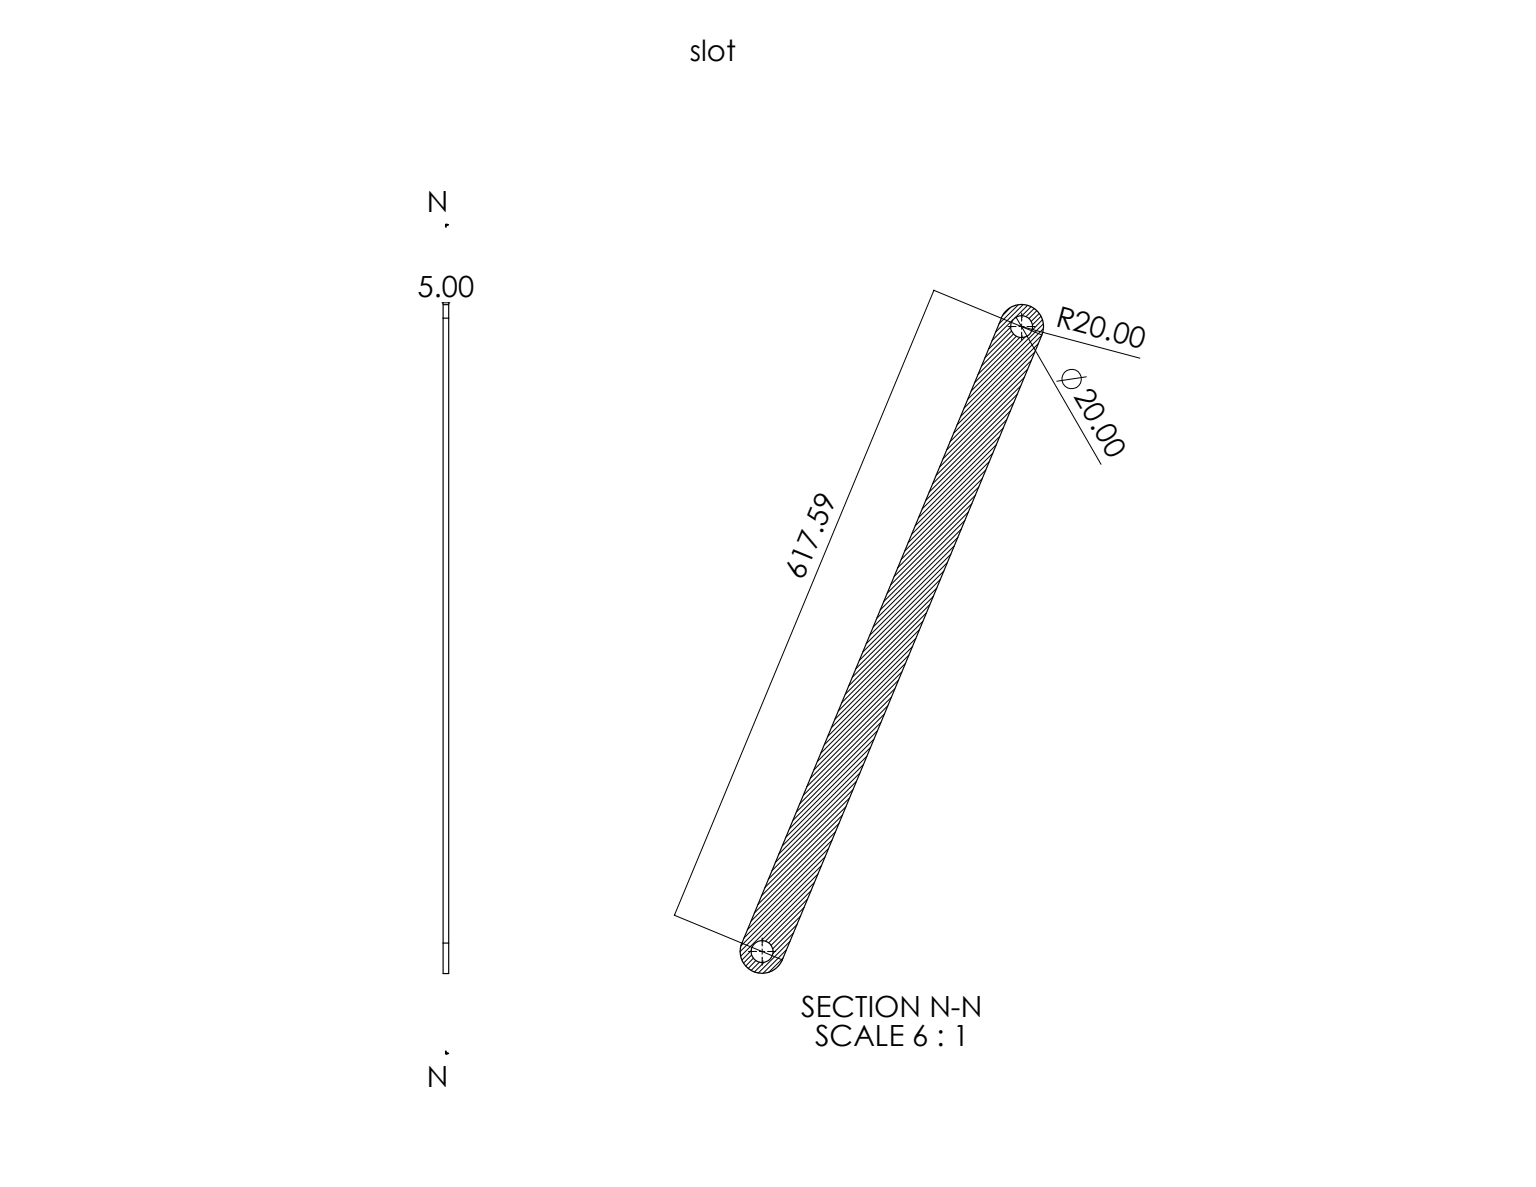
ISO-10303-21;
HEADER;
FILE_DESCRIPTION (('STEP AP214'),
    '1' );
FILE_NAME ('Slot.step',
    '2026-10-21T17:07:05',
    ( '' ),
    ( '' ),
    'SwSTEP 2.0',
    'SolidWorks 2025',
    '' );
FILE_SCHEMA (( 'AUTOMOTIVE_DESIGN' ));
ENDSEC;

DATA;
#41=DIRECTION ( 'NONE',  ( 1.000000000000000000, 0.000000000000000000, 0.000000000000000000 ) ) ;
#52=CYLINDRICAL_SURFACE ( 'NONE', #32876, 9.999999999999980460 ) ;
#346=VERTEX_POINT ( 'NONE', #30093 ) ;
#367=EDGE_LOOP ( 'NONE', ( #42116, #38302, #12349, #11045 ) ) ;
#472=ORIENTED_EDGE ( 'NONE', *, *, #31485, .F. ) ;
#592=ORIENTED_EDGE ( 'NONE', *, *, #31485, .T. ) ;
#799=EDGE_LOOP ( 'NONE', ( #25522, #592, #42461, #2264, #39166 ) ) ;
#822=CARTESIAN_POINT ( 'NONE',  ( 799.9999999999993179, 205.0000000000000568, -255.0000000000000000 ) ) ;
#930=CIRCLE ( 'NONE', #36312, 10.00000000000000888 ) ;
#1035=CIRCLE ( 'NONE', #26827, 20.00000000000004619 ) ;
#1068=VECTOR ( 'NONE', #44629, 1000.000000000000000 ) ;
#1080=EDGE_LOOP ( 'NONE', ( #33357, #6990 ) ) ;
#1302=DIRECTION ( 'NONE',  ( 1.000000000000000000, 0.000000000000000000, 0.000000000000000000 ) ) ;
#1372=DIRECTION ( 'NONE',  ( 0.000000000000000000, 0.000000000000000000, -1.000000000000000000 ) ) ;
#1425=ORIENTED_EDGE ( 'NONE', *, *, #20505, .T. ) ;
#1710=CYLINDRICAL_SURFACE ( 'NONE', #21162, 9.999999999999982236 ) ;
#1788=EDGE_CURVE ( 'NONE', #28471, #16704, #1035, .T. ) ;
#1790=VECTOR ( 'NONE', #5422, 1000.000000000000000 ) ;
#1945=DIRECTION ( 'NONE',  ( -1.000000000000000000, -0.000000000000000000, -0.000000000000000000 ) ) ;
#1955=EDGE_CURVE ( 'NONE', #29157, #346, #26860, .T. ) ;
#2029=ORIENTED_EDGE ( 'NONE', *, *, #37278, .F. ) ;
#2061=EDGE_CURVE ( 'NONE', #2904, #27191, #30531, .T. ) ;
#2125=CIRCLE ( 'NONE', #8059, 20.00000000000004619 ) ;
#2238=ORIENTED_EDGE ( 'NONE', *, *, #32386, .T. ) ;
#2241=DIRECTION ( 'NONE',  ( -1.000000000000000000, -0.000000000000000000, -0.000000000000000000 ) ) ;
#2264=ORIENTED_EDGE ( 'NONE', *, *, #37278, .T. ) ;
#2415=EDGE_CURVE ( 'NONE', #35075, #33515, #40175, .T. ) ;
#2494=LINE ( 'NONE', #37839, #35001 ) ;
#2512=CARTESIAN_POINT ( 'NONE',  ( 799.9999999999993179, 205.0000000000000568, -255.0000000000000000 ) ) ;
#2552=ORIENTED_EDGE ( 'NONE', *, *, #44509, .T. ) ;
#2733=DIRECTION ( 'NONE',  ( -1.000000000000000000, -0.000000000000000000, -0.000000000000000000 ) ) ;
#2774=DIRECTION ( 'NONE',  ( -1.000000000000000000, -0.000000000000000000, -0.000000000000000000 ) ) ;
#2904=VERTEX_POINT ( 'NONE', #22866 ) ;
#2983=FACE_OUTER_BOUND ( 'NONE', #799, .T. ) ;
#3048=CARTESIAN_POINT ( 'NONE',  ( 799.9999999999993179, -365.3551492539851893, -18.13243251470705886 ) ) ;
#3132=ORIENTED_EDGE ( 'NONE', *, *, #28735, .F. ) ;
#3295=CIRCLE ( 'NONE', #4026, 9.999999999999980460 ) ;
#3590=DIRECTION ( 'NONE',  ( -1.000000000000000000, -0.000000000000000000, -0.000000000000000000 ) ) ;
#4011=DIRECTION ( 'NONE',  ( 0.000000000000000000, 0.000000000000000000, 1.000000000000000000 ) ) ;
#4026=AXIS2_PLACEMENT_3D ( 'NONE', #19087, #1302, #25779 ) ;
#4037=VERTEX_POINT ( 'NONE', #18447 ) ;
#4474=CYLINDRICAL_SURFACE ( 'NONE', #18007, 9.999999999999980460 ) ;
#4695=DIRECTION ( 'NONE',  ( 1.000000000000000000, 0.000000000000000000, 0.000000000000000000 ) ) ;
#4728=AXIS2_PLACEMENT_3D ( 'NONE', #30831, #20871, #44925 ) ;
#4975=LINE ( 'NONE', #37049, #24120 ) ;
#5041=CARTESIAN_POINT ( 'NONE',  ( 799.9999999999993179, -365.3551492539851893, -18.13243251470705886 ) ) ;
#5166=UNCERTAINTY_MEASURE_WITH_UNIT (LENGTH_MEASURE( 1.000000000000000082E-05 ), #31589, 'distance_accuracy_value', 'NONE');
#5422=DIRECTION ( 'NONE',  ( -1.000000000000000000, -0.000000000000000000, -0.000000000000000000 ) ) ;
#5439=ORIENTED_EDGE ( 'NONE', *, *, #32681, .F. ) ;
#5952=LINE ( 'NONE', #12438, #14488 ) ;
#5959=CARTESIAN_POINT ( 'NONE',  ( 799.9999999999993179, -365.3551492539851893, -18.13243251470705886 ) ) ;
#5960=ORIENTED_EDGE ( 'NONE', *, *, #32681, .T. ) ;
#6047=CARTESIAN_POINT ( 'NONE',  ( 794.9999999999993179, 205.0000000000000568, -255.0000000000000000 ) ) ;
#6075=DIRECTION ( 'NONE',  ( 1.000000000000000000, 0.000000000000000000, 0.000000000000000000 ) ) ;
#6630=ADVANCED_FACE ( 'NONE', ( #25717 ), #15099, .T. ) ;
#6645=CARTESIAN_POINT ( 'NONE',  ( 799.9999999999993179, -373.0259173205825505, -36.60293108048681887 ) ) ;
#6755=ORIENTED_EDGE ( 'NONE', *, *, #8285, .F. ) ;
#6971=DIRECTION ( 'NONE',  ( 1.000000000000000000, 0.000000000000000000, 0.000000000000000000 ) ) ;
#6990=ORIENTED_EDGE ( 'NONE', *, *, #41635, .F. ) ;
#6992=CIRCLE ( 'NONE', #15147, 9.999999999999980460 ) ;
#7095=DIRECTION ( 'NONE',  ( 0.000000000000000000, 0.000000000000000000, -1.000000000000000000 ) ) ;
#7396=EDGE_LOOP ( 'NONE', ( #39858, #16678, #2238, #24707 ) ) ;
#7535=DIRECTION ( 'NONE',  ( -1.000000000000000000, -0.000000000000000000, -0.000000000000000000 ) ) ;
#7734=CLOSED_SHELL ( 'NONE', ( #18555, #27777, #6630, #41065, #10811, #12974, #23831, #28874, #36584, #32049, #44130 ) ) ;
#7743=AXIS2_PLACEMENT_3D ( 'NONE', #32884, #18571, #14660 ) ;
#7832=DIRECTION ( 'NONE',  ( 1.000000000000000000, 0.000000000000000000, 0.000000000000000000 ) ) ;
#7854=CARTESIAN_POINT ( 'NONE',  ( 794.9999999999993179, 197.3292319334027241, -273.4704985657796783 ) ) ;
#7892=ORIENTED_EDGE ( 'NONE', *, *, #20407, .T. ) ;
#7941=ORIENTED_EDGE ( 'NONE', *, *, #2415, .F. ) ;
#8020=PLANE ( 'NONE',  #45644 ) ;
#8059=AXIS2_PLACEMENT_3D ( 'NONE', #3048, #10428, #24747 ) ;
#8089=CARTESIAN_POINT ( 'NONE',  ( 799.9999999999993179, 205.0000000000000568, -255.0000000000000000 ) ) ;
#8162=DIRECTION ( 'NONE',  ( 0.000000000000000000, 0.000000000000000000, -1.000000000000000000 ) ) ;
#8190=ORIENTED_EDGE ( 'NONE', *, *, #44419, .F. ) ;
#8211=ORIENTED_EDGE ( 'NONE', *, *, #32386, .F. ) ;
#8219=DIRECTION ( 'NONE',  ( 0.000000000000000000, 0.000000000000000000, -1.000000000000000000 ) ) ;
#8278=VECTOR ( 'NONE', #32707, 1000.000000000000114 ) ;
#8285=EDGE_CURVE ( 'NONE', #28471, #35075, #20083, .T. ) ;
#8538=CYLINDRICAL_SURFACE ( 'NONE', #43823, 20.00000000000004974 ) ;
#8579=STYLED_ITEM('',(#45758),#32652);
#8682=DIRECTION ( 'NONE',  ( -1.000000000000000000, -0.000000000000000000, -0.000000000000000000 ) ) ;
#8705=ORIENTED_EDGE ( 'NONE', *, *, #27181, .F. ) ;
#9439=FACE_OUTER_BOUND ( 'NONE', #367, .T. ) ;
#9490=AXIS2_PLACEMENT_3D ( 'NONE', #31456, #41, #42544 ) ;
#9501=ORIENTED_EDGE ( 'NONE', *, *, #22196, .T. ) ;
#9722=SHAPE_DEFINITION_REPRESENTATION ( #12958, #26911 ) ;
#9827=CARTESIAN_POINT ( 'NONE',  ( 794.9999999999993179, -365.3551492539851893, 1.867567485292990437 ) ) ;
#9866=AXIS2_PLACEMENT_3D ( 'NONE', #20927, #14026, #28095 ) ;
#9886=ORIENTED_EDGE ( 'NONE', *, *, #15887, .T. ) ;
#10366=ORIENTED_EDGE ( 'NONE', *, *, #28918, .F. ) ;
#10428=DIRECTION ( 'NONE',  ( 1.000000000000000000, 0.000000000000000000, 0.000000000000000000 ) ) ;
#10454=EDGE_LOOP ( 'NONE', ( #9886, #8705, #24590, #5960 ) ) ;
#10811=ADVANCED_FACE ( 'NONE', ( #19673, #29404, #15538 ), #19007, .F. ) ;
#11045=ORIENTED_EDGE ( 'NONE', *, *, #2415, .T. ) ;
#11116=CARTESIAN_POINT ( 'NONE',  ( 799.9999999999993179, 212.6707680665973612, -236.5295014342203785 ) ) ;
#11406=AXIS2_PLACEMENT_3D ( 'NONE', #40174, #12225, #1372 ) ;
#11479=CARTESIAN_POINT ( 'NONE',  ( 799.9999999999993179, 197.3292319334027241, -273.4704985657796783 ) ) ;
#11636=CARTESIAN_POINT ( 'NONE',  ( 799.9999999999993179, -365.3551492539851893, 1.867567485292990437 ) ) ;
#11665=VERTEX_POINT ( 'NONE', #36674 ) ;
#11901=CARTESIAN_POINT ( 'NONE',  ( 794.9999999999993179, 205.0000000000000568, -265.0000000000000000 ) ) ;
#12099=LINE ( 'NONE', #43723, #33619 ) ;
#12225=DIRECTION ( 'NONE',  ( 1.000000000000000000, 0.000000000000000000, 0.000000000000000000 ) ) ;
#12335=ORIENTED_EDGE ( 'NONE', *, *, #32641, .T. ) ;
#12349=ORIENTED_EDGE ( 'NONE', *, *, #8285, .T. ) ;
#12384=DIRECTION ( 'NONE',  ( 0.000000000000000000, 0.000000000000000000, -1.000000000000000000 ) ) ;
#12438=CARTESIAN_POINT ( 'NONE',  ( 799.9999999999993179, -365.3551492539851893, -28.13243251470704109 ) ) ;
#12675=VERTEX_POINT ( 'NONE', #25969 ) ;
#12762=DIRECTION ( 'NONE',  ( 0.000000000000000000, -0.9235249282889854694, 0.3835384033298675499 ) ) ;
#12874=FACE_OUTER_BOUND ( 'NONE', #32634, .T. ) ;
#12915=EDGE_LOOP ( 'NONE', ( #45177, #30430, #8190, #7941, #26500 ) ) ;
#12923=AXIS2_PLACEMENT_3D ( 'NONE', #36384, #39878, #8219 ) ;
#12958=PRODUCT_DEFINITION_SHAPE ( 'NONE', 'NONE',  #21378 ) ;
#12974=ADVANCED_FACE ( 'NONE', ( #14922 ), #39185, .T. ) ;
#12976=ORIENTED_EDGE ( 'NONE', *, *, #20505, .F. ) ;
#12990=AXIS2_PLACEMENT_3D ( 'NONE', #36612, #40071, #44208 ) ;
#13478=( NAMED_UNIT ( * ) PLANE_ANGLE_UNIT ( ) SI_UNIT ( $, .RADIAN. ) );
#13724=PRODUCT ( 'Slot', 'Slot', '', ( #16662 ) ) ;
#13829=ORIENTED_EDGE ( 'NONE', *, *, #32525, .F. ) ;
#13973=EDGE_CURVE ( 'NONE', #37595, #38147, #14651, .T. ) ;
#14026=DIRECTION ( 'NONE',  ( 1.000000000000000000, 0.000000000000000000, 0.000000000000000000 ) ) ;
#14045=DIRECTION ( 'NONE',  ( -1.000000000000000000, -0.000000000000000000, -0.000000000000000000 ) ) ;
#14295=APPLICATION_CONTEXT ( 'automotive_design' ) ;
#14488=VECTOR ( 'NONE', #2733, 1000.000000000000000 ) ;
#14651=LINE ( 'NONE', #26323, #34401 ) ;
#14660=DIRECTION ( 'NONE',  ( 0.000000000000000000, 0.000000000000000000, 1.000000000000000000 ) ) ;
#14890=CARTESIAN_POINT ( 'NONE',  ( 799.9999999999993179, -365.3551492539851893, -28.13243251470704109 ) ) ;
#14922=FACE_OUTER_BOUND ( 'NONE', #26806, .T. ) ;
#15099=CYLINDRICAL_SURFACE ( 'NONE', #7743, 20.00000000000004974 ) ;
#15147=AXIS2_PLACEMENT_3D ( 'NONE', #44707, #29697, #12384 ) ;
#15222=DIRECTION ( 'NONE',  ( 1.000000000000000000, 0.000000000000000000, 0.000000000000000000 ) ) ;
#15538=FACE_BOUND ( 'NONE', #16425, .T. ) ;
#15887=EDGE_CURVE ( 'NONE', #31020, #29157, #36625, .T. ) ;
#16425=EDGE_LOOP ( 'NONE', ( #36307, #2552 ) ) ;
#16617=DIRECTION ( 'NONE',  ( 0.000000000000000000, 0.000000000000000000, -1.000000000000000000 ) ) ;
#16662=PRODUCT_CONTEXT ( 'NONE', #20748, 'mechanical' ) ;
#16678=ORIENTED_EDGE ( 'NONE', *, *, #41635, .T. ) ;
#16704=VERTEX_POINT ( 'NONE', #11636 ) ;
#16905=ORIENTED_EDGE ( 'NONE', *, *, #2061, .T. ) ;
#17509=ORIENTED_EDGE ( 'NONE', *, *, #32525, .T. ) ;
#17814=VERTEX_POINT ( 'NONE', #11116 ) ;
#17930=PRODUCT_DEFINITION_FORMATION_WITH_SPECIFIED_SOURCE ( 'ANY', '', #13724, .NOT_KNOWN. ) ;
#18007=AXIS2_PLACEMENT_3D ( 'NONE', #18565, #39597, #4011 ) ;
#18368=CARTESIAN_POINT ( 'NONE',  ( 794.9999999999993179, -373.0259173205825505, -36.60293108048681887 ) ) ;
#18447=CARTESIAN_POINT ( 'NONE',  ( 794.9999999999993179, -365.3551492539851893, -8.132432514707076621 ) ) ;
#18450=DIRECTION ( 'NONE',  ( 0.000000000000000000, 0.000000000000000000, -1.000000000000000000 ) ) ;
#18478=FACE_OUTER_BOUND ( 'NONE', #7396, .T. ) ;
#18555=ADVANCED_FACE ( 'NONE', ( #33159 ), #1710, .F. ) ;
#18565=CARTESIAN_POINT ( 'NONE',  ( 799.9999999999993179, 205.0000000000000568, -255.0000000000000000 ) ) ;
#18571=DIRECTION ( 'NONE',  ( -1.000000000000000000, -0.000000000000000000, -0.000000000000000000 ) ) ;
#18664=EDGE_CURVE ( 'NONE', #27191, #35548, #30722, .T. ) ;
#18864=CARTESIAN_POINT ( 'NONE',  ( 799.9999999999993179, -365.3551492539851893, -8.132432514707076621 ) ) ;
#18922=AXIS2_PLACEMENT_3D ( 'NONE', #33307, #29619, #8162 ) ;
#19007=PLANE ( 'NONE',  #18922 ) ;
#19087=CARTESIAN_POINT ( 'NONE',  ( 799.9999999999993179, -365.3551492539851893, -18.13243251470705886 ) ) ;
#19488=PLANE ( 'NONE',  #12990 ) ;
#19673=FACE_OUTER_BOUND ( 'NONE', #12915, .T. ) ;
#20083=LINE ( 'NONE', #27254, #21008 ) ;
#20279=EDGE_LOOP ( 'NONE', ( #36315, #16905, #41774, #8211 ) ) ;
#20394=( LENGTH_UNIT ( ) NAMED_UNIT ( * ) SI_UNIT ( .MILLI., .METRE. ) );
#20407=EDGE_CURVE ( 'NONE', #38193, #4037, #23195, .T. ) ;
#20505=EDGE_CURVE ( 'NONE', #38193, #21185, #3295, .T. ) ;
#20748=APPLICATION_CONTEXT ( 'automotive_design' ) ;
#20871=DIRECTION ( 'NONE',  ( 1.000000000000000000, 0.000000000000000000, 0.000000000000000000 ) ) ;
#20927=CARTESIAN_POINT ( 'NONE',  ( 794.9999999999993179, -365.3551492539851893, -18.13243251470705886 ) ) ;
#21008=VECTOR ( 'NONE', #2774, 1000.000000000000000 ) ;
#21162=AXIS2_PLACEMENT_3D ( 'NONE', #29248, #8682, #32705 ) ;
#21185=VERTEX_POINT ( 'NONE', #14890 ) ;
#21378=PRODUCT_DEFINITION ( 'UNKNOWN', '', #17930, #23776 ) ;
#21631=EDGE_CURVE ( 'NONE', #21185, #38193, #6992, .T. ) ;
#21701=( GEOMETRIC_REPRESENTATION_CONTEXT ( 3 ) GLOBAL_UNCERTAINTY_ASSIGNED_CONTEXT ( ( #21814 ) ) GLOBAL_UNIT_ASSIGNED_CONTEXT ( ( #20394, #13478, #41652 ) ) REPRESENTATION_CONTEXT ( 'NONE', 'WORKASPACE' ) );
#21814=UNCERTAINTY_MEASURE_WITH_UNIT (LENGTH_MEASURE( 1.000000000000000082E-05 ), #20394, 'distance_accuracy_value', 'NONE');
#21866=DIRECTION ( 'NONE',  ( -0.000000000000000000, 0.3835384033298669948, 0.9235249282889858025 ) ) ;
#22062=FACE_OUTER_BOUND ( 'NONE', #26478, .T. ) ;
#22076=CARTESIAN_POINT ( 'NONE',  ( 794.9999999999993179, 197.3292319334027241, -273.4704985657796783 ) ) ;
#22196=EDGE_CURVE ( 'NONE', #16704, #33515, #37771, .T. ) ;
#22441=ORIENTED_EDGE ( 'NONE', *, *, #1955, .T. ) ;
#22463=CARTESIAN_POINT ( 'NONE',  ( 799.9999999999993179, -365.3551492539851893, -18.13243251470705886 ) ) ;
#22569=VECTOR ( 'NONE', #14045, 1000.000000000000000 ) ;
#22822=LINE ( 'NONE', #6645, #22569 ) ;
#22866=CARTESIAN_POINT ( 'NONE',  ( 799.9999999999993179, 205.0000000000000568, -265.0000000000000000 ) ) ;
#23096=AXIS2_PLACEMENT_3D ( 'NONE', #38282, #31785, #7095 ) ;
#23153=CARTESIAN_POINT ( 'NONE',  ( 0.000000000000000000, 0.000000000000000000, 0.000000000000000000 ) ) ;
#23195=LINE ( 'NONE', #18864, #1790 ) ;
#23764=CARTESIAN_POINT ( 'NONE',  ( 799.9999999999993179, 197.3292319334027241, -273.4704985657796783 ) ) ;
#23776=PRODUCT_DEFINITION_CONTEXT ( 'detailed design', #14295, 'design' ) ;
#23831=ADVANCED_FACE ( 'NONE', ( #22062 ), #19488, .F. ) ;
#24120=VECTOR ( 'NONE', #1945, 1000.000000000000000 ) ;
#24252=CARTESIAN_POINT ( 'NONE',  ( 794.9999999999993179, 205.0000000000000568, -245.0000000000000284 ) ) ;
#24492=AXIS2_PLACEMENT_3D ( 'NONE', #2512, #45027, #16617 ) ;
#24521=ORIENTED_EDGE ( 'NONE', *, *, #45346, .T. ) ;
#24590=ORIENTED_EDGE ( 'NONE', *, *, #13973, .F. ) ;
#24662=AXIS2_PLACEMENT_3D ( 'NONE', #6047, #26164, #33547 ) ;
#24707=ORIENTED_EDGE ( 'NONE', *, *, #18664, .F. ) ;
#24747=DIRECTION ( 'NONE',  ( 0.000000000000000000, 0.000000000000000000, -1.000000000000000000 ) ) ;
#24856=AXIS2_PLACEMENT_3D ( 'NONE', #39712, #7832, #18450 ) ;
#24973=CIRCLE ( 'NONE', #9490, 10.00000000000000888 ) ;
#25193=CARTESIAN_POINT ( 'NONE',  ( 799.9999999999993179, -373.0259173205825505, -36.60293108048681887 ) ) ;
#25522=ORIENTED_EDGE ( 'NONE', *, *, #28735, .T. ) ;
#25717=FACE_OUTER_BOUND ( 'NONE', #25837, .T. ) ;
#25779=DIRECTION ( 'NONE',  ( 0.000000000000000000, 0.000000000000000000, -1.000000000000000000 ) ) ;
#25787=EDGE_CURVE ( 'NONE', #4037, #12675, #29295, .T. ) ;
#25837=EDGE_LOOP ( 'NONE', ( #2029, #9501, #29733, #5439 ) ) ;
#25957=ORIENTED_EDGE ( 'NONE', *, *, #25787, .F. ) ;
#25969=CARTESIAN_POINT ( 'NONE',  ( 794.9999999999993179, -365.3551492539851893, -28.13243251470704109 ) ) ;
#26063=DIRECTION ( 'NONE',  ( 0.000000000000000000, 0.000000000000000000, 1.000000000000000000 ) ) ;
#26071=CIRCLE ( 'NONE', #9866, 9.999999999999980460 ) ;
#26164=DIRECTION ( 'NONE',  ( 1.000000000000000000, 0.000000000000000000, 0.000000000000000000 ) ) ;
#26323=CARTESIAN_POINT ( 'NONE',  ( 799.9999999999993179, 197.3292319334027241, -273.4704985657796783 ) ) ;
#26342=CARTESIAN_POINT ( 'NONE',  ( 799.9999999999993179, -365.3551492539851893, -8.132432514707076621 ) ) ;
#26393=CARTESIAN_POINT ( 'NONE',  ( 799.9999999999993179, 205.0000000000000568, -265.0000000000000000 ) ) ;
#26478=EDGE_LOOP ( 'NONE', ( #12335, #6755, #472, #37362 ) ) ;
#26500=ORIENTED_EDGE ( 'NONE', *, *, #32641, .F. ) ;
#26806=EDGE_LOOP ( 'NONE', ( #22441, #10366, #3132, #33771 ) ) ;
#26827=AXIS2_PLACEMENT_3D ( 'NONE', #22463, #4695, #36571 ) ;
#26858=AXIS2_PLACEMENT_3D ( 'NONE', #23153, #34241, #6075 ) ;
#26860=CIRCLE ( 'NONE', #24662, 19.99999999999990763 ) ;
#26911=SHAPE_REPRESENTATION ( 'Slot', ( #26858 ), #21701 ) ;
#26977=DIRECTION ( 'NONE',  ( 0.000000000000000000, -0.9235249282889854694, 0.3835384033298675499 ) ) ;
#27007=PLANE ( 'NONE',  #24492 ) ;
#27181=EDGE_CURVE ( 'NONE', #38147, #29157, #4975, .T. ) ;
#27191=VERTEX_POINT ( 'NONE', #11901 ) ;
#27254=CARTESIAN_POINT ( 'NONE',  ( 799.9999999999993179, -357.6843811873878280, 0.3380660510726891665 ) ) ;
#27278=ORIENTED_EDGE ( 'NONE', *, *, #20407, .F. ) ;
#27777=ADVANCED_FACE ( 'NONE', ( #35882 ), #4474, .F. ) ;
#28095=DIRECTION ( 'NONE',  ( 0.000000000000000000, 0.000000000000000000, -1.000000000000000000 ) ) ;
#28251=AXIS2_PLACEMENT_3D ( 'NONE', #5041, #2241, #44286 ) ;
#28471=VERTEX_POINT ( 'NONE', #32343 ) ;
#28472=SHAPE_REPRESENTATION_RELATIONSHIP ( 'NONE' , 'NONE' ,  #26911, #32092 ) ;
#28536=EDGE_LOOP ( 'NONE', ( #24521, #32241 ) ) ;
#28574=DIRECTION ( 'NONE',  ( 0.000000000000000000, -0.9235249282889858025, 0.3835384033298669948 ) ) ;
#28735=EDGE_CURVE ( 'NONE', #38147, #17814, #29113, .T. ) ;
#28874=ADVANCED_FACE ( 'NONE', ( #9439 ), #8538, .T. ) ;
#28918=EDGE_CURVE ( 'NONE', #17814, #346, #2494, .T. ) ;
#28923=ORIENTED_EDGE ( 'NONE', *, *, #21631, .T. ) ;
#29113=CIRCLE ( 'NONE', #11406, 19.99999999999990763 ) ;
#29157=VERTEX_POINT ( 'NONE', #7854 ) ;
#29186=VECTOR ( 'NONE', #3590, 1000.000000000000000 ) ;
#29248=CARTESIAN_POINT ( 'NONE',  ( 799.9999999999993179, -365.3551492539851893, -18.13243251470705886 ) ) ;
#29252=AXIS2_PLACEMENT_3D ( 'NONE', #822, #7535, #39872 ) ;
#29295=CIRCLE ( 'NONE', #24856, 9.999999999999980460 ) ;
#29334=DIRECTION ( 'NONE',  ( 0.000000000000000000, 0.000000000000000000, 1.000000000000000000 ) ) ;
#29404=FACE_BOUND ( 'NONE', #28536, .T. ) ;
#29619=DIRECTION ( 'NONE',  ( 1.000000000000000000, 0.000000000000000000, 0.000000000000000000 ) ) ;
#29662=ORIENTED_EDGE ( 'NONE', *, *, #44509, .F. ) ;
#29697=DIRECTION ( 'NONE',  ( 1.000000000000000000, 0.000000000000000000, 0.000000000000000000 ) ) ;
#29733=ORIENTED_EDGE ( 'NONE', *, *, #44419, .T. ) ;
#30093=CARTESIAN_POINT ( 'NONE',  ( 794.9999999999993179, 212.6707680665973612, -236.5295014342203785 ) ) ;
#30430=ORIENTED_EDGE ( 'NONE', *, *, #15887, .F. ) ;
#30456=FACE_BOUND ( 'NONE', #1080, .T. ) ;
#30531=LINE ( 'NONE', #26393, #1068 ) ;
#30722=CIRCLE ( 'NONE', #12923, 10.00000000000000888 ) ;
#30831=CARTESIAN_POINT ( 'NONE',  ( 794.9999999999993179, 205.0000000000000568, -255.0000000000000000 ) ) ;
#31020=VERTEX_POINT ( 'NONE', #18368 ) ;
#31444=MECHANICAL_DESIGN_GEOMETRIC_PRESENTATION_REPRESENTATION('',(#8579),#38817);
#31454=CARTESIAN_POINT ( 'NONE',  ( 794.9999999999993179, -365.3551492539851893, -18.13243251470705886 ) ) ;
#31456=CARTESIAN_POINT ( 'NONE',  ( 799.9999999999993179, 205.0000000000000568, -255.0000000000000000 ) ) ;
#31485=EDGE_CURVE ( 'NONE', #17814, #28471, #12099, .T. ) ;
#31589=( LENGTH_UNIT ( ) NAMED_UNIT ( * ) SI_UNIT ( .MILLI., .METRE. ) );
#31671=DIRECTION ( 'NONE',  ( 0.000000000000000000, 0.000000000000000000, -1.000000000000000000 ) ) ;
#31785=DIRECTION ( 'NONE',  ( 1.000000000000000000, 0.000000000000000000, 0.000000000000000000 ) ) ;
#32049=ADVANCED_FACE ( 'NONE', ( #18478 ), #52, .F. ) ;
#32092=ADVANCED_BREP_SHAPE_REPRESENTATION ( '', ( #32652, #26858 ), #21701 ) ;
#32241=ORIENTED_EDGE ( 'NONE', *, *, #18664, .T. ) ;
#32343=CARTESIAN_POINT ( 'NONE',  ( 799.9999999999993179, -357.6843811873878280, 0.3380660510726891665 ) ) ;
#32386=EDGE_CURVE ( 'NONE', #11665, #35548, #41077, .T. ) ;
#32525=EDGE_CURVE ( 'NONE', #21185, #12675, #5952, .T. ) ;
#32634=EDGE_LOOP ( 'NONE', ( #13829, #28923, #7892, #29662 ) ) ;
#32641=EDGE_CURVE ( 'NONE', #346, #35075, #37831, .T. ) ;
#32652=MANIFOLD_SOLID_BREP ( 'Boss-Extrude21', #7734 ) ;
#32681=EDGE_CURVE ( 'NONE', #37595, #31020, #22822, .T. ) ;
#32705=DIRECTION ( 'NONE',  ( 0.000000000000000000, 0.000000000000000000, 1.000000000000000000 ) ) ;
#32707=DIRECTION ( 'NONE',  ( -0.000000000000000000, 0.9235249282889856914, -0.3835384033298670503 ) ) ;
#32876=AXIS2_PLACEMENT_3D ( 'NONE', #8089, #36467, #29334 ) ;
#32884=CARTESIAN_POINT ( 'NONE',  ( 799.9999999999993179, -365.3551492539851893, -18.13243251470705886 ) ) ;
#33159=FACE_OUTER_BOUND ( 'NONE', #35410, .T. ) ;
#33232=ORIENTED_EDGE ( 'NONE', *, *, #21631, .F. ) ;
#33307=CARTESIAN_POINT ( 'NONE',  ( 794.9999999999993179, 205.0000000000000568, -255.0000000000000000 ) ) ;
#33357=ORIENTED_EDGE ( 'NONE', *, *, #37373, .F. ) ;
#33424=DIRECTION ( 'NONE',  ( 0.000000000000000000, 0.000000000000000000, -1.000000000000000000 ) ) ;
#33515=VERTEX_POINT ( 'NONE', #9827 ) ;
#33547=DIRECTION ( 'NONE',  ( 0.000000000000000000, 0.000000000000000000, -1.000000000000000000 ) ) ;
#33619=VECTOR ( 'NONE', #12762, 1000.000000000000114 ) ;
#33771=ORIENTED_EDGE ( 'NONE', *, *, #27181, .T. ) ;
#33888=CYLINDRICAL_SURFACE ( 'NONE', #28251, 9.999999999999982236 ) ;
#34141=FACE_BOUND ( 'NONE', #39350, .T. ) ;
#34241=DIRECTION ( 'NONE',  ( 0.000000000000000000, 0.000000000000000000, 1.000000000000000000 ) ) ;
#34362=CARTESIAN_POINT ( 'NONE',  ( 794.9999999999993179, 212.6707680665973612, -236.5295014342203785 ) ) ;
#34401=VECTOR ( 'NONE', #39129, 1000.000000000000114 ) ;
#35001=VECTOR ( 'NONE', #44786, 1000.000000000000000 ) ;
#35075=VERTEX_POINT ( 'NONE', #38885 ) ;
#35215=CARTESIAN_POINT ( 'NONE',  ( 799.9999999999993179, -365.3551492539851893, 1.867567485292990437 ) ) ;
#35274=( NAMED_UNIT ( * ) PLANE_ANGLE_UNIT ( ) SI_UNIT ( $, .RADIAN. ) );
#35410=EDGE_LOOP ( 'NONE', ( #1425, #17509, #25957, #27278 ) ) ;
#35548=VERTEX_POINT ( 'NONE', #24252 ) ;
#35882=FACE_OUTER_BOUND ( 'NONE', #20279, .T. ) ;
#36307=ORIENTED_EDGE ( 'NONE', *, *, #25787, .T. ) ;
#36312=AXIS2_PLACEMENT_3D ( 'NONE', #40141, #15222, #33424 ) ;
#36315=ORIENTED_EDGE ( 'NONE', *, *, #37373, .T. ) ;
#36384=CARTESIAN_POINT ( 'NONE',  ( 794.9999999999993179, 205.0000000000000568, -255.0000000000000000 ) ) ;
#36467=DIRECTION ( 'NONE',  ( -1.000000000000000000, -0.000000000000000000, -0.000000000000000000 ) ) ;
#36571=DIRECTION ( 'NONE',  ( 0.000000000000000000, 0.000000000000000000, -1.000000000000000000 ) ) ;
#36584=ADVANCED_FACE ( 'NONE', ( #42878 ), #8020, .F. ) ;
#36612=CARTESIAN_POINT ( 'NONE',  ( 799.9999999999993179, 212.6707680665973612, -236.5295014342203785 ) ) ;
#36625=LINE ( 'NONE', #22076, #8278 ) ;
#36674=CARTESIAN_POINT ( 'NONE',  ( 799.9999999999993179, 205.0000000000000568, -245.0000000000000284 ) ) ;
#37049=CARTESIAN_POINT ( 'NONE',  ( 799.9999999999993179, 197.3292319334027241, -273.4704985657796783 ) ) ;
#37278=EDGE_CURVE ( 'NONE', #16704, #37595, #2125, .T. ) ;
#37362=ORIENTED_EDGE ( 'NONE', *, *, #28918, .T. ) ;
#37373=EDGE_CURVE ( 'NONE', #11665, #2904, #24973, .T. ) ;
#37595=VERTEX_POINT ( 'NONE', #25193 ) ;
#37771=LINE ( 'NONE', #35215, #29186 ) ;
#37831=LINE ( 'NONE', #34362, #42497 ) ;
#37839=CARTESIAN_POINT ( 'NONE',  ( 799.9999999999993179, 212.6707680665973612, -236.5295014342203785 ) ) ;
#38147=VERTEX_POINT ( 'NONE', #23764 ) ;
#38193=VERTEX_POINT ( 'NONE', #26342 ) ;
#38282=CARTESIAN_POINT ( 'NONE',  ( 794.9999999999993179, -365.3551492539851893, -18.13243251470705886 ) ) ;
#38302=ORIENTED_EDGE ( 'NONE', *, *, #1788, .F. ) ;
#38817=( GEOMETRIC_REPRESENTATION_CONTEXT ( 3 ) GLOBAL_UNCERTAINTY_ASSIGNED_CONTEXT ( ( #5166 ) ) GLOBAL_UNIT_ASSIGNED_CONTEXT ( ( #31589, #35274, #45217 ) ) REPRESENTATION_CONTEXT ( 'NONE', 'WORKASPACE' ) );
#38885=CARTESIAN_POINT ( 'NONE',  ( 794.9999999999993179, -357.6843811873878280, 0.3380660510726891665 ) ) ;
#39129=DIRECTION ( 'NONE',  ( -0.000000000000000000, 0.9235249282889856914, -0.3835384033298670503 ) ) ;
#39166=ORIENTED_EDGE ( 'NONE', *, *, #13973, .T. ) ;
#39185=CYLINDRICAL_SURFACE ( 'NONE', #29252, 19.99999999999990763 ) ;
#39350=EDGE_LOOP ( 'NONE', ( #12976, #33232 ) ) ;
#39436=AXIS2_PLACEMENT_3D ( 'NONE', #31454, #6971, #31671 ) ;
#39597=DIRECTION ( 'NONE',  ( -1.000000000000000000, -0.000000000000000000, -0.000000000000000000 ) ) ;
#39712=CARTESIAN_POINT ( 'NONE',  ( 794.9999999999993179, -365.3551492539851893, -18.13243251470705886 ) ) ;
#39858=ORIENTED_EDGE ( 'NONE', *, *, #2061, .F. ) ;
#39872=DIRECTION ( 'NONE',  ( 0.000000000000000000, 0.000000000000000000, 1.000000000000000000 ) ) ;
#39878=DIRECTION ( 'NONE',  ( 1.000000000000000000, 0.000000000000000000, 0.000000000000000000 ) ) ;
#40071=DIRECTION ( 'NONE',  ( 0.000000000000000000, -0.3835384033298676054, -0.9235249282889855804 ) ) ;
#40141=CARTESIAN_POINT ( 'NONE',  ( 799.9999999999993179, 205.0000000000000568, -255.0000000000000000 ) ) ;
#40174=CARTESIAN_POINT ( 'NONE',  ( 799.9999999999993179, 205.0000000000000568, -255.0000000000000000 ) ) ;
#40175=CIRCLE ( 'NONE', #39436, 20.00000000000004619 ) ;
#40857=CIRCLE ( 'NONE', #4728, 10.00000000000000888 ) ;
#41065=ADVANCED_FACE ( 'NONE', ( #30456, #2983, #34141 ), #27007, .T. ) ;
#41077=LINE ( 'NONE', #41305, #45471 ) ;
#41305=CARTESIAN_POINT ( 'NONE',  ( 799.9999999999993179, 205.0000000000000568, -245.0000000000000284 ) ) ;
#41635=EDGE_CURVE ( 'NONE', #2904, #11665, #930, .T. ) ;
#41652=( NAMED_UNIT ( * ) SI_UNIT ( $, .STERADIAN. ) SOLID_ANGLE_UNIT ( ) );
#41774=ORIENTED_EDGE ( 'NONE', *, *, #45346, .F. ) ;
#42116=ORIENTED_EDGE ( 'NONE', *, *, #22196, .F. ) ;
#42461=ORIENTED_EDGE ( 'NONE', *, *, #1788, .T. ) ;
#42497=VECTOR ( 'NONE', #26977, 1000.000000000000114 ) ;
#42544=DIRECTION ( 'NONE',  ( 0.000000000000000000, 0.000000000000000000, -1.000000000000000000 ) ) ;
#42878=FACE_OUTER_BOUND ( 'NONE', #10454, .T. ) ;
#43038=CIRCLE ( 'NONE', #23096, 20.00000000000004619 ) ;
#43630=DIRECTION ( 'NONE',  ( -1.000000000000000000, -0.000000000000000000, -0.000000000000000000 ) ) ;
#43723=CARTESIAN_POINT ( 'NONE',  ( 799.9999999999993179, 212.6707680665973612, -236.5295014342203785 ) ) ;
#43823=AXIS2_PLACEMENT_3D ( 'NONE', #5959, #43630, #26063 ) ;
#44130=ADVANCED_FACE ( 'NONE', ( #12874 ), #33888, .F. ) ;
#44208=DIRECTION ( 'NONE',  ( 0.000000000000000000, 0.9235249282889854694, -0.3835384033298675499 ) ) ;
#44286=DIRECTION ( 'NONE',  ( 0.000000000000000000, 0.000000000000000000, 1.000000000000000000 ) ) ;
#44302=DIRECTION ( 'NONE',  ( -1.000000000000000000, -0.000000000000000000, -0.000000000000000000 ) ) ;
#44419=EDGE_CURVE ( 'NONE', #33515, #31020, #43038, .T. ) ;
#44509=EDGE_CURVE ( 'NONE', #12675, #4037, #26071, .T. ) ;
#44629=DIRECTION ( 'NONE',  ( -1.000000000000000000, -0.000000000000000000, -0.000000000000000000 ) ) ;
#44707=CARTESIAN_POINT ( 'NONE',  ( 799.9999999999993179, -365.3551492539851893, -18.13243251470705886 ) ) ;
#44786=DIRECTION ( 'NONE',  ( -1.000000000000000000, -0.000000000000000000, -0.000000000000000000 ) ) ;
#44925=DIRECTION ( 'NONE',  ( 0.000000000000000000, 0.000000000000000000, -1.000000000000000000 ) ) ;
#45027=DIRECTION ( 'NONE',  ( 1.000000000000000000, 0.000000000000000000, 0.000000000000000000 ) ) ;
#45177=ORIENTED_EDGE ( 'NONE', *, *, #1955, .F. ) ;
#45217=( NAMED_UNIT ( * ) SI_UNIT ( $, .STERADIAN. ) SOLID_ANGLE_UNIT ( ) );
#45346=EDGE_CURVE ( 'NONE', #35548, #27191, #40857, .T. ) ;
#45471=VECTOR ( 'NONE', #44302, 1000.000000000000000 ) ;
#45644=AXIS2_PLACEMENT_3D ( 'NONE', #11479, #21866, #28574 ) ;
#45752=COLOUR_RGB('Sky Blue',0.24,0.69,0.87);
#45753=FILL_AREA_STYLE_COLOUR('',#45752);
#45754=FILL_AREA_STYLE('',(#45753));
#45755=SURFACE_STYLE_FILL_AREA(#45754);
#45756=SURFACE_SIDE_STYLE('',(#45755));
#45757=SURFACE_STYLE_USAGE(.BOTH.,#45756);
#45758=PRESENTATION_STYLE_ASSIGNMENT((#45757));
ENDSEC;
END-ISO-10303-21;
